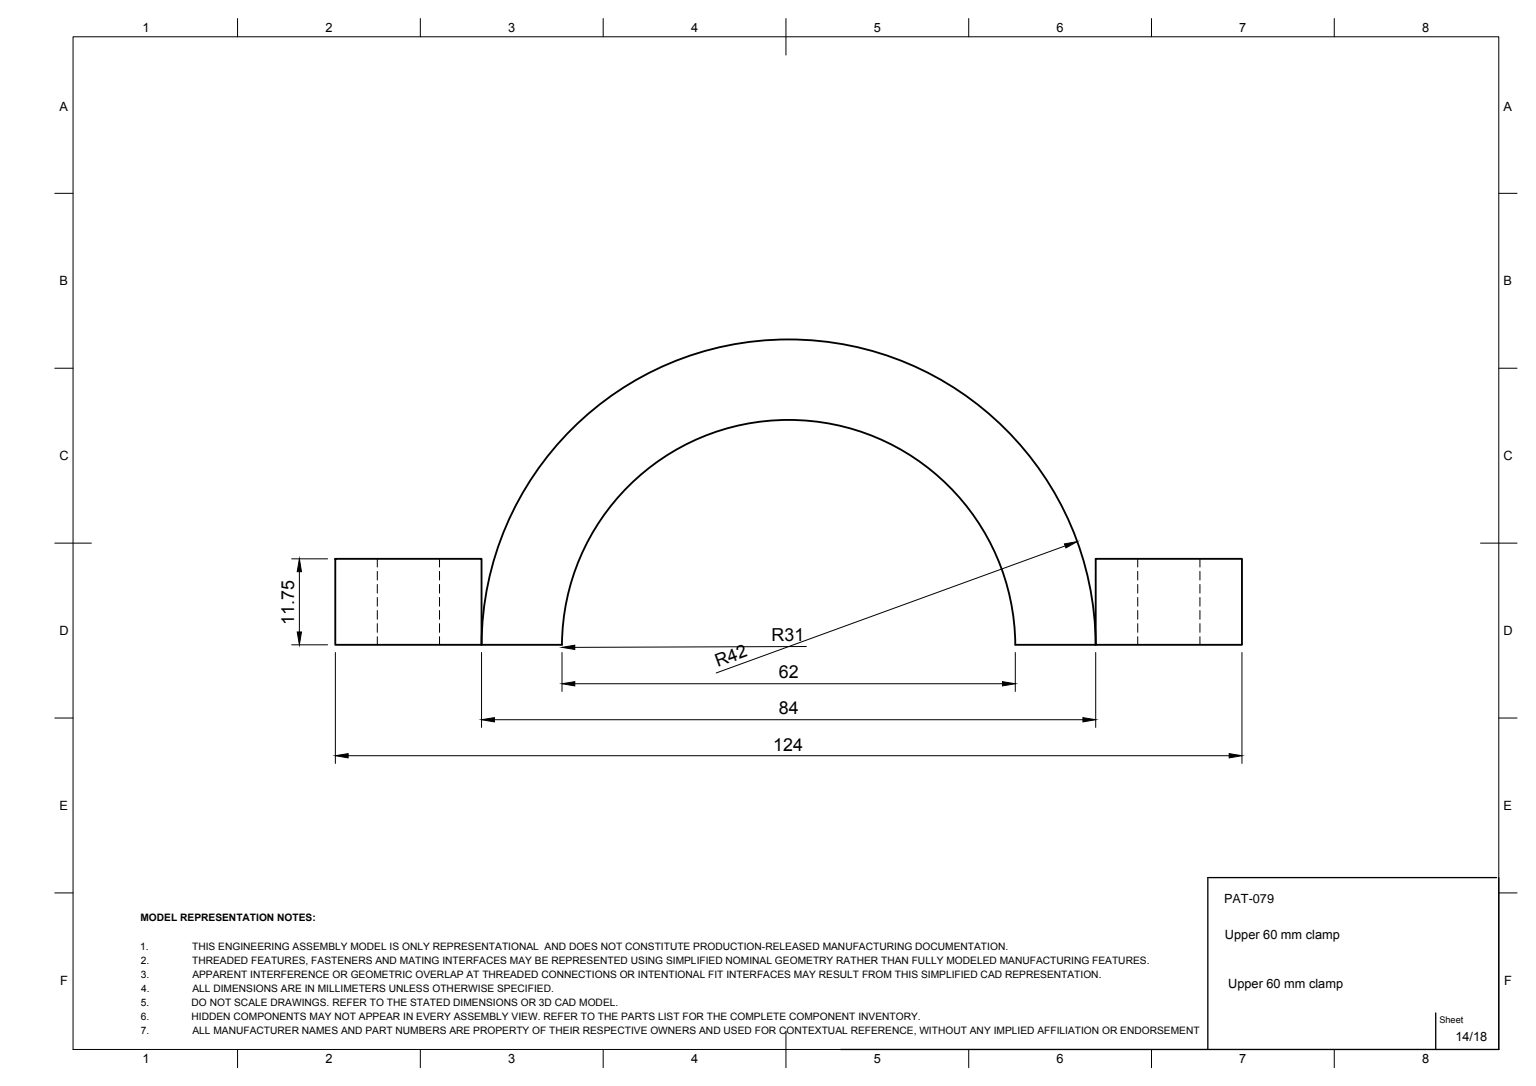
ISO-10303-21;
HEADER;
/* Generated by software containing ST-Developer
 * from STEP Tools, Inc. (www.steptools.com) 
 */

FILE_DESCRIPTION(
/* description */ ('Pipe clamp stand with threaded column'),
/* implementation_level */ '2;1');

FILE_NAME(
/* name */ 'Upper 60 mm clamp.step',
/* time_stamp */ '2026-10-27T10:55:48-07:00',
/* author */ (''),
/* organization */ (''),
/* preprocessor_version */ 'ST-DEVELOPER v20.2',
/* originating_system */ 'Autodesk Translation Framework v15.17.0.0',
/* authorisation */ '');

FILE_SCHEMA (('AUTOMOTIVE_DESIGN { 1 0 10303 214 3 1 1 }'));
ENDSEC;

DATA;
#10=MECHANICAL_DESIGN_GEOMETRIC_PRESENTATION_REPRESENTATION('',(#756,#757,#758),#34433);
#706=SHAPE_REPRESENTATION_RELATIONSHIP('SRR','None',#34548,#728);
#728=ADVANCED_BREP_SHAPE_REPRESENTATION('',(#786,#787,#788),#34416);
#756=STYLED_ITEM('',(#34729),#786);
#757=STYLED_ITEM('',(#34729),#787);
#758=STYLED_ITEM('',(#34729),#788);
#786=MANIFOLD_SOLID_BREP('Body1',#8783);
#787=MANIFOLD_SOLID_BREP('Body2',#8784);
#788=MANIFOLD_SOLID_BREP('Body3',#8785);
#838=FACE_BOUND('',#1893,.T.);
#839=FACE_BOUND('',#1896,.T.);
#840=FACE_BOUND('',#1902,.T.);
#841=FACE_BOUND('',#1905,.T.);
#943=PLANE('',#9448);
#944=PLANE('',#9450);
#945=PLANE('',#9451);
#946=PLANE('',#9454);
#947=PLANE('',#9458);
#948=PLANE('',#9459);
#949=PLANE('',#9460);
#950=PLANE('',#9461);
#951=PLANE('',#9462);
#952=PLANE('',#9463);
#953=PLANE('',#9467);
#954=PLANE('',#9468);
#955=PLANE('',#9469);
#956=PLANE('',#9470);
#957=PLANE('',#9471);
#958=PLANE('',#9472);
#1358=FACE_OUTER_BOUND('',#1884,.T.);
#1359=FACE_OUTER_BOUND('',#1885,.T.);
#1360=FACE_OUTER_BOUND('',#1886,.T.);
#1361=FACE_OUTER_BOUND('',#1887,.T.);
#1362=FACE_OUTER_BOUND('',#1888,.T.);
#1363=FACE_OUTER_BOUND('',#1889,.T.);
#1364=FACE_OUTER_BOUND('',#1890,.T.);
#1365=FACE_OUTER_BOUND('',#1891,.T.);
#1366=FACE_OUTER_BOUND('',#1892,.T.);
#1367=FACE_OUTER_BOUND('',#1894,.T.);
#1368=FACE_OUTER_BOUND('',#1895,.T.);
#1369=FACE_OUTER_BOUND('',#1897,.T.);
#1370=FACE_OUTER_BOUND('',#1898,.T.);
#1371=FACE_OUTER_BOUND('',#1899,.T.);
#1372=FACE_OUTER_BOUND('',#1900,.T.);
#1373=FACE_OUTER_BOUND('',#1901,.T.);
#1374=FACE_OUTER_BOUND('',#1903,.T.);
#1375=FACE_OUTER_BOUND('',#1904,.T.);
#1376=FACE_OUTER_BOUND('',#1906,.T.);
#1377=FACE_OUTER_BOUND('',#1907,.T.);
#1884=EDGE_LOOP('',(#7199,#7200,#7201,#7202));
#1885=EDGE_LOOP('',(#7203,#7204,#7205,#7206));
#1886=EDGE_LOOP('',(#7207,#7208,#7209,#7210));
#1887=EDGE_LOOP('',(#7211,#7212,#7213,#7214));
#1888=EDGE_LOOP('',(#7215,#7216,#7217,#7218));
#1889=EDGE_LOOP('',(#7219,#7220,#7221,#7222));
#1890=EDGE_LOOP('',(#7223,#7224,#7225,#7226));
#1891=EDGE_LOOP('',(#7227,#7228,#7229,#7230));
#1892=EDGE_LOOP('',(#7231,#7232,#7233,#7234));
#1893=EDGE_LOOP('',(#7235));
#1894=EDGE_LOOP('',(#7236,#7237,#7238,#7239));
#1895=EDGE_LOOP('',(#7240,#7241,#7242,#7243));
#1896=EDGE_LOOP('',(#7244));
#1897=EDGE_LOOP('',(#7245,#7246,#7247,#7248));
#1898=EDGE_LOOP('',(#7249,#7250,#7251,#7252));
#1899=EDGE_LOOP('',(#7253,#7254,#7255,#7256));
#1900=EDGE_LOOP('',(#7257,#7258,#7259,#7260));
#1901=EDGE_LOOP('',(#7261,#7262,#7263,#7264));
#1902=EDGE_LOOP('',(#7265));
#1903=EDGE_LOOP('',(#7266,#7267,#7268,#7269));
#1904=EDGE_LOOP('',(#7270,#7271,#7272,#7273));
#1905=EDGE_LOOP('',(#7274));
#1906=EDGE_LOOP('',(#7275,#7276,#7277,#7278));
#1907=EDGE_LOOP('',(#7279,#7280,#7281,#7282));
#2457=LINE('',#28483,#3074);
#2458=LINE('',#28487,#3075);
#2459=LINE('',#28491,#3076);
#2460=LINE('',#28494,#3077);
#2461=LINE('',#28497,#3078);
#2462=LINE('',#28498,#3079);
#2463=LINE('',#28501,#3080);
#2464=LINE('',#28502,#3081);
#2465=LINE('',#28510,#3082);
#2466=LINE('',#28515,#3083);
#2467=LINE('',#28517,#3084);
#2468=LINE('',#28519,#3085);
#2469=LINE('',#28520,#3086);
#2470=LINE('',#28523,#3087);
#2471=LINE('',#28525,#3088);
#2472=LINE('',#28526,#3089);
#2473=LINE('',#28529,#3090);
#2474=LINE('',#28531,#3091);
#2475=LINE('',#28532,#3092);
#2476=LINE('',#28534,#3093);
#2477=LINE('',#28535,#3094);
#2478=LINE('',#28542,#3095);
#2479=LINE('',#28547,#3096);
#2480=LINE('',#28549,#3097);
#2481=LINE('',#28551,#3098);
#2482=LINE('',#28552,#3099);
#2483=LINE('',#28555,#3100);
#2484=LINE('',#28557,#3101);
#2485=LINE('',#28558,#3102);
#2486=LINE('',#28561,#3103);
#2487=LINE('',#28563,#3104);
#2488=LINE('',#28564,#3105);
#2489=LINE('',#28566,#3106);
#2490=LINE('',#28567,#3107);
#3074=VECTOR('',#10912,1.);
#3075=VECTOR('',#10915,1.);
#3076=VECTOR('',#10920,1.);
#3077=VECTOR('',#10923,1.);
#3078=VECTOR('',#10926,1.);
#3079=VECTOR('',#10927,1.);
#3080=VECTOR('',#10930,1.);
#3081=VECTOR('',#10931,1.);
#3082=VECTOR('',#10942,0.425);
#3083=VECTOR('',#10947,1.);
#3084=VECTOR('',#10948,1.);
#3085=VECTOR('',#10949,1.);
#3086=VECTOR('',#10950,1.);
#3087=VECTOR('',#10953,1.);
#3088=VECTOR('',#10954,1.);
#3089=VECTOR('',#10955,1.);
#3090=VECTOR('',#10958,1.);
#3091=VECTOR('',#10959,1.);
#3092=VECTOR('',#10960,1.);
#3093=VECTOR('',#10963,1.);
#3094=VECTOR('',#10964,1.);
#3095=VECTOR('',#10973,0.425);
#3096=VECTOR('',#10978,1.);
#3097=VECTOR('',#10979,1.);
#3098=VECTOR('',#10980,1.);
#3099=VECTOR('',#10981,1.);
#3100=VECTOR('',#10984,1.);
#3101=VECTOR('',#10985,1.);
#3102=VECTOR('',#10986,1.);
#3103=VECTOR('',#10989,1.);
#3104=VECTOR('',#10990,1.);
#3105=VECTOR('',#10991,1.);
#3106=VECTOR('',#10994,1.);
#3107=VECTOR('',#10995,1.);
#3388=CIRCLE('',#9446,3.1);
#3389=CIRCLE('',#9447,3.1);
#3390=CIRCLE('',#9449,4.2);
#3391=CIRCLE('',#9453,4.2);
#3392=CIRCLE('',#9456,0.425);
#3393=CIRCLE('',#9457,0.425);
#3394=CIRCLE('',#9465,0.425);
#3395=CIRCLE('',#9466,0.425);
#4006=VERTEX_POINT('',#28481);
#4007=VERTEX_POINT('',#28482);
#4008=VERTEX_POINT('',#28484);
#4009=VERTEX_POINT('',#28486);
#4010=VERTEX_POINT('',#28490);
#4011=VERTEX_POINT('',#28492);
#4012=VERTEX_POINT('',#28496);
#4013=VERTEX_POINT('',#28500);
#4014=VERTEX_POINT('',#28507);
#4015=VERTEX_POINT('',#28509);
#4016=VERTEX_POINT('',#28513);
#4017=VERTEX_POINT('',#28514);
#4018=VERTEX_POINT('',#28516);
#4019=VERTEX_POINT('',#28518);
#4020=VERTEX_POINT('',#28522);
#4021=VERTEX_POINT('',#28524);
#4022=VERTEX_POINT('',#28528);
#4023=VERTEX_POINT('',#28530);
#4024=VERTEX_POINT('',#28539);
#4025=VERTEX_POINT('',#28541);
#4026=VERTEX_POINT('',#28545);
#4027=VERTEX_POINT('',#28546);
#4028=VERTEX_POINT('',#28548);
#4029=VERTEX_POINT('',#28550);
#4030=VERTEX_POINT('',#28554);
#4031=VERTEX_POINT('',#28556);
#4032=VERTEX_POINT('',#28560);
#4033=VERTEX_POINT('',#28562);
#5113=EDGE_CURVE('',#4006,#4007,#2457,.T.);
#5114=EDGE_CURVE('',#4008,#4006,#3388,.T.);
#5115=EDGE_CURVE('',#4009,#4008,#2458,.T.);
#5116=EDGE_CURVE('',#4007,#4009,#3389,.T.);
#5117=EDGE_CURVE('',#4006,#4010,#2459,.T.);
#5118=EDGE_CURVE('',#4010,#4011,#3390,.T.);
#5119=EDGE_CURVE('',#4011,#4008,#2460,.T.);
#5120=EDGE_CURVE('',#4012,#4007,#2461,.T.);
#5121=EDGE_CURVE('',#4010,#4012,#2462,.T.);
#5122=EDGE_CURVE('',#4013,#4011,#2463,.T.);
#5123=EDGE_CURVE('',#4009,#4013,#2464,.T.);
#5124=EDGE_CURVE('',#4012,#4013,#3391,.T.);
#5125=EDGE_CURVE('',#4014,#4014,#3392,.T.);
#5126=EDGE_CURVE('',#4014,#4015,#2465,.T.);
#5127=EDGE_CURVE('',#4015,#4015,#3393,.T.);
#5128=EDGE_CURVE('',#4016,#4017,#2466,.T.);
#5129=EDGE_CURVE('',#4016,#4018,#2467,.T.);
#5130=EDGE_CURVE('',#4019,#4018,#2468,.T.);
#5131=EDGE_CURVE('',#4017,#4019,#2469,.T.);
#5132=EDGE_CURVE('',#4017,#4020,#2470,.T.);
#5133=EDGE_CURVE('',#4021,#4019,#2471,.T.);
#5134=EDGE_CURVE('',#4020,#4021,#2472,.T.);
#5135=EDGE_CURVE('',#4020,#4022,#2473,.T.);
#5136=EDGE_CURVE('',#4023,#4021,#2474,.T.);
#5137=EDGE_CURVE('',#4022,#4023,#2475,.T.);
#5138=EDGE_CURVE('',#4022,#4016,#2476,.T.);
#5139=EDGE_CURVE('',#4018,#4023,#2477,.T.);
#5140=EDGE_CURVE('',#4024,#4024,#3394,.T.);
#5141=EDGE_CURVE('',#4024,#4025,#2478,.T.);
#5142=EDGE_CURVE('',#4025,#4025,#3395,.T.);
#5143=EDGE_CURVE('',#4026,#4027,#2479,.T.);
#5144=EDGE_CURVE('',#4026,#4028,#2480,.T.);
#5145=EDGE_CURVE('',#4029,#4028,#2481,.T.);
#5146=EDGE_CURVE('',#4027,#4029,#2482,.T.);
#5147=EDGE_CURVE('',#4027,#4030,#2483,.T.);
#5148=EDGE_CURVE('',#4031,#4029,#2484,.T.);
#5149=EDGE_CURVE('',#4030,#4031,#2485,.T.);
#5150=EDGE_CURVE('',#4030,#4032,#2486,.T.);
#5151=EDGE_CURVE('',#4033,#4031,#2487,.T.);
#5152=EDGE_CURVE('',#4032,#4033,#2488,.T.);
#5153=EDGE_CURVE('',#4032,#4026,#2489,.T.);
#5154=EDGE_CURVE('',#4028,#4033,#2490,.T.);
#7199=ORIENTED_EDGE('',*,*,#5113,.F.);
#7200=ORIENTED_EDGE('',*,*,#5114,.F.);
#7201=ORIENTED_EDGE('',*,*,#5115,.F.);
#7202=ORIENTED_EDGE('',*,*,#5116,.F.);
#7203=ORIENTED_EDGE('',*,*,#5114,.T.);
#7204=ORIENTED_EDGE('',*,*,#5117,.T.);
#7205=ORIENTED_EDGE('',*,*,#5118,.T.);
#7206=ORIENTED_EDGE('',*,*,#5119,.T.);
#7207=ORIENTED_EDGE('',*,*,#5113,.T.);
#7208=ORIENTED_EDGE('',*,*,#5120,.F.);
#7209=ORIENTED_EDGE('',*,*,#5121,.F.);
#7210=ORIENTED_EDGE('',*,*,#5117,.F.);
#7211=ORIENTED_EDGE('',*,*,#5115,.T.);
#7212=ORIENTED_EDGE('',*,*,#5119,.F.);
#7213=ORIENTED_EDGE('',*,*,#5122,.F.);
#7214=ORIENTED_EDGE('',*,*,#5123,.F.);
#7215=ORIENTED_EDGE('',*,*,#5122,.T.);
#7216=ORIENTED_EDGE('',*,*,#5118,.F.);
#7217=ORIENTED_EDGE('',*,*,#5121,.T.);
#7218=ORIENTED_EDGE('',*,*,#5124,.T.);
#7219=ORIENTED_EDGE('',*,*,#5116,.T.);
#7220=ORIENTED_EDGE('',*,*,#5123,.T.);
#7221=ORIENTED_EDGE('',*,*,#5124,.F.);
#7222=ORIENTED_EDGE('',*,*,#5120,.T.);
#7223=ORIENTED_EDGE('',*,*,#5125,.F.);
#7224=ORIENTED_EDGE('',*,*,#5126,.T.);
#7225=ORIENTED_EDGE('',*,*,#5127,.F.);
#7226=ORIENTED_EDGE('',*,*,#5126,.F.);
#7227=ORIENTED_EDGE('',*,*,#5128,.F.);
#7228=ORIENTED_EDGE('',*,*,#5129,.T.);
#7229=ORIENTED_EDGE('',*,*,#5130,.F.);
#7230=ORIENTED_EDGE('',*,*,#5131,.F.);
#7231=ORIENTED_EDGE('',*,*,#5132,.F.);
#7232=ORIENTED_EDGE('',*,*,#5131,.T.);
#7233=ORIENTED_EDGE('',*,*,#5133,.F.);
#7234=ORIENTED_EDGE('',*,*,#5134,.F.);
#7235=ORIENTED_EDGE('',*,*,#5125,.T.);
#7236=ORIENTED_EDGE('',*,*,#5135,.F.);
#7237=ORIENTED_EDGE('',*,*,#5134,.T.);
#7238=ORIENTED_EDGE('',*,*,#5136,.F.);
#7239=ORIENTED_EDGE('',*,*,#5137,.F.);
#7240=ORIENTED_EDGE('',*,*,#5138,.F.);
#7241=ORIENTED_EDGE('',*,*,#5137,.T.);
#7242=ORIENTED_EDGE('',*,*,#5139,.F.);
#7243=ORIENTED_EDGE('',*,*,#5129,.F.);
#7244=ORIENTED_EDGE('',*,*,#5127,.T.);
#7245=ORIENTED_EDGE('',*,*,#5139,.T.);
#7246=ORIENTED_EDGE('',*,*,#5136,.T.);
#7247=ORIENTED_EDGE('',*,*,#5133,.T.);
#7248=ORIENTED_EDGE('',*,*,#5130,.T.);
#7249=ORIENTED_EDGE('',*,*,#5138,.T.);
#7250=ORIENTED_EDGE('',*,*,#5128,.T.);
#7251=ORIENTED_EDGE('',*,*,#5132,.T.);
#7252=ORIENTED_EDGE('',*,*,#5135,.T.);
#7253=ORIENTED_EDGE('',*,*,#5140,.F.);
#7254=ORIENTED_EDGE('',*,*,#5141,.T.);
#7255=ORIENTED_EDGE('',*,*,#5142,.F.);
#7256=ORIENTED_EDGE('',*,*,#5141,.F.);
#7257=ORIENTED_EDGE('',*,*,#5143,.F.);
#7258=ORIENTED_EDGE('',*,*,#5144,.T.);
#7259=ORIENTED_EDGE('',*,*,#5145,.F.);
#7260=ORIENTED_EDGE('',*,*,#5146,.F.);
#7261=ORIENTED_EDGE('',*,*,#5147,.F.);
#7262=ORIENTED_EDGE('',*,*,#5146,.T.);
#7263=ORIENTED_EDGE('',*,*,#5148,.F.);
#7264=ORIENTED_EDGE('',*,*,#5149,.F.);
#7265=ORIENTED_EDGE('',*,*,#5140,.T.);
#7266=ORIENTED_EDGE('',*,*,#5150,.F.);
#7267=ORIENTED_EDGE('',*,*,#5149,.T.);
#7268=ORIENTED_EDGE('',*,*,#5151,.F.);
#7269=ORIENTED_EDGE('',*,*,#5152,.F.);
#7270=ORIENTED_EDGE('',*,*,#5153,.F.);
#7271=ORIENTED_EDGE('',*,*,#5152,.T.);
#7272=ORIENTED_EDGE('',*,*,#5154,.F.);
#7273=ORIENTED_EDGE('',*,*,#5144,.F.);
#7274=ORIENTED_EDGE('',*,*,#5142,.T.);
#7275=ORIENTED_EDGE('',*,*,#5154,.T.);
#7276=ORIENTED_EDGE('',*,*,#5151,.T.);
#7277=ORIENTED_EDGE('',*,*,#5148,.T.);
#7278=ORIENTED_EDGE('',*,*,#5145,.T.);
#7279=ORIENTED_EDGE('',*,*,#5153,.T.);
#7280=ORIENTED_EDGE('',*,*,#5143,.T.);
#7281=ORIENTED_EDGE('',*,*,#5147,.T.);
#7282=ORIENTED_EDGE('',*,*,#5150,.T.);
#8225=CYLINDRICAL_SURFACE('',#9445,3.1);
#8226=CYLINDRICAL_SURFACE('',#9452,4.2);
#8227=CYLINDRICAL_SURFACE('',#9455,0.425);
#8228=CYLINDRICAL_SURFACE('',#9464,0.425);
#8595=ADVANCED_FACE('',(#1358),#8225,.F.);
#8596=ADVANCED_FACE('',(#1359),#943,.T.);
#8597=ADVANCED_FACE('',(#1360),#944,.F.);
#8598=ADVANCED_FACE('',(#1361),#945,.F.);
#8599=ADVANCED_FACE('',(#1362),#8226,.T.);
#8600=ADVANCED_FACE('',(#1363),#946,.F.);
#8601=ADVANCED_FACE('',(#1364),#8227,.F.);
#8602=ADVANCED_FACE('',(#1365),#947,.T.);
#8603=ADVANCED_FACE('',(#1366,#838),#948,.T.);
#8604=ADVANCED_FACE('',(#1367),#949,.T.);
#8605=ADVANCED_FACE('',(#1368,#839),#950,.T.);
#8606=ADVANCED_FACE('',(#1369),#951,.T.);
#8607=ADVANCED_FACE('',(#1370),#952,.F.);
#8608=ADVANCED_FACE('',(#1371),#8228,.F.);
#8609=ADVANCED_FACE('',(#1372),#953,.T.);
#8610=ADVANCED_FACE('',(#1373,#840),#954,.T.);
#8611=ADVANCED_FACE('',(#1374),#955,.T.);
#8612=ADVANCED_FACE('',(#1375,#841),#956,.T.);
#8613=ADVANCED_FACE('',(#1376),#957,.T.);
#8614=ADVANCED_FACE('',(#1377),#958,.F.);
#8783=CLOSED_SHELL('',(#8595,#8596,#8597,#8598,#8599,#8600));
#8784=CLOSED_SHELL('',(#8601,#8602,#8603,#8604,#8605,#8606,#8607));
#8785=CLOSED_SHELL('',(#8608,#8609,#8610,#8611,#8612,#8613,#8614));
#9444=AXIS2_PLACEMENT_3D('',#28479,#10908,#10909);
#9445=AXIS2_PLACEMENT_3D('',#28480,#10910,#10911);
#9446=AXIS2_PLACEMENT_3D('',#28485,#10913,#10914);
#9447=AXIS2_PLACEMENT_3D('',#28488,#10916,#10917);
#9448=AXIS2_PLACEMENT_3D('',#28489,#10918,#10919);
#9449=AXIS2_PLACEMENT_3D('',#28493,#10921,#10922);
#9450=AXIS2_PLACEMENT_3D('',#28495,#10924,#10925);
#9451=AXIS2_PLACEMENT_3D('',#28499,#10928,#10929);
#9452=AXIS2_PLACEMENT_3D('',#28503,#10932,#10933);
#9453=AXIS2_PLACEMENT_3D('',#28504,#10934,#10935);
#9454=AXIS2_PLACEMENT_3D('',#28505,#10936,#10937);
#9455=AXIS2_PLACEMENT_3D('',#28506,#10938,#10939);
#9456=AXIS2_PLACEMENT_3D('',#28508,#10940,#10941);
#9457=AXIS2_PLACEMENT_3D('',#28511,#10943,#10944);
#9458=AXIS2_PLACEMENT_3D('',#28512,#10945,#10946);
#9459=AXIS2_PLACEMENT_3D('',#28521,#10951,#10952);
#9460=AXIS2_PLACEMENT_3D('',#28527,#10956,#10957);
#9461=AXIS2_PLACEMENT_3D('',#28533,#10961,#10962);
#9462=AXIS2_PLACEMENT_3D('',#28536,#10965,#10966);
#9463=AXIS2_PLACEMENT_3D('',#28537,#10967,#10968);
#9464=AXIS2_PLACEMENT_3D('',#28538,#10969,#10970);
#9465=AXIS2_PLACEMENT_3D('',#28540,#10971,#10972);
#9466=AXIS2_PLACEMENT_3D('',#28543,#10974,#10975);
#9467=AXIS2_PLACEMENT_3D('',#28544,#10976,#10977);
#9468=AXIS2_PLACEMENT_3D('',#28553,#10982,#10983);
#9469=AXIS2_PLACEMENT_3D('',#28559,#10987,#10988);
#9470=AXIS2_PLACEMENT_3D('',#28565,#10992,#10993);
#9471=AXIS2_PLACEMENT_3D('',#28568,#10996,#10997);
#9472=AXIS2_PLACEMENT_3D('',#28569,#10998,#10999);
#10908=DIRECTION('axis',(0.,0.,1.));
#10909=DIRECTION('refdir',(1.,0.,0.));
#10910=DIRECTION('center_axis',(0.,1.,0.));
#10911=DIRECTION('ref_axis',(1.,0.,0.));
#10912=DIRECTION('',(0.,-1.,0.));
#10913=DIRECTION('center_axis',(0.,-1.,0.));
#10914=DIRECTION('ref_axis',(1.,0.,0.));
#10915=DIRECTION('',(0.,1.,0.));
#10916=DIRECTION('center_axis',(0.,1.,0.));
#10917=DIRECTION('ref_axis',(1.,0.,0.));
#10918=DIRECTION('center_axis',(0.,1.,0.));
#10919=DIRECTION('ref_axis',(1.,0.,0.));
#10920=DIRECTION('',(-1.,0.,0.));
#10921=DIRECTION('center_axis',(0.,1.,0.));
#10922=DIRECTION('ref_axis',(1.,0.,0.));
#10923=DIRECTION('',(-1.,0.,0.));
#10924=DIRECTION('center_axis',(0.,0.,1.));
#10925=DIRECTION('ref_axis',(1.,0.,0.));
#10926=DIRECTION('',(1.,0.,0.));
#10927=DIRECTION('',(0.,-1.,0.));
#10928=DIRECTION('center_axis',(0.,0.,1.));
#10929=DIRECTION('ref_axis',(1.,0.,0.));
#10930=DIRECTION('',(0.,1.,0.));
#10931=DIRECTION('',(1.,0.,0.));
#10932=DIRECTION('center_axis',(0.,1.,0.));
#10933=DIRECTION('ref_axis',(1.,0.,0.));
#10934=DIRECTION('center_axis',(0.,1.,0.));
#10935=DIRECTION('ref_axis',(1.,0.,0.));
#10936=DIRECTION('center_axis',(0.,1.,0.));
#10937=DIRECTION('ref_axis',(1.,0.,0.));
#10938=DIRECTION('center_axis',(0.,0.,1.));
#10939=DIRECTION('ref_axis',(1.,0.,0.));
#10940=DIRECTION('center_axis',(0.,0.,1.));
#10941=DIRECTION('ref_axis',(1.,0.,0.));
#10942=DIRECTION('',(0.,0.,1.));
#10943=DIRECTION('center_axis',(0.,0.,-1.));
#10944=DIRECTION('ref_axis',(1.,0.,0.));
#10945=DIRECTION('center_axis',(-1.,0.,0.));
#10946=DIRECTION('ref_axis',(0.,0.,1.));
#10947=DIRECTION('',(0.,0.,-1.));
#10948=DIRECTION('',(0.,1.,0.));
#10949=DIRECTION('',(0.,0.,1.));
#10950=DIRECTION('',(0.,1.,0.));
#10951=DIRECTION('center_axis',(0.,0.,-1.));
#10952=DIRECTION('ref_axis',(-1.,0.,0.));
#10953=DIRECTION('',(1.,0.,0.));
#10954=DIRECTION('',(-1.,0.,0.));
#10955=DIRECTION('',(0.,1.,0.));
#10956=DIRECTION('center_axis',(1.,0.,0.));
#10957=DIRECTION('ref_axis',(0.,0.,-1.));
#10958=DIRECTION('',(0.,0.,1.));
#10959=DIRECTION('',(0.,0.,-1.));
#10960=DIRECTION('',(0.,1.,0.));
#10961=DIRECTION('center_axis',(0.,0.,1.));
#10962=DIRECTION('ref_axis',(1.,0.,0.));
#10963=DIRECTION('',(-1.,0.,0.));
#10964=DIRECTION('',(1.,0.,0.));
#10965=DIRECTION('center_axis',(0.,1.,0.));
#10966=DIRECTION('ref_axis',(0.,0.,1.));
#10967=DIRECTION('center_axis',(0.,1.,0.));
#10968=DIRECTION('ref_axis',(1.,0.,0.));
#10969=DIRECTION('center_axis',(0.,0.,1.));
#10970=DIRECTION('ref_axis',(1.,0.,0.));
#10971=DIRECTION('center_axis',(0.,0.,1.));
#10972=DIRECTION('ref_axis',(1.,0.,0.));
#10973=DIRECTION('',(0.,0.,1.));
#10974=DIRECTION('center_axis',(0.,0.,-1.));
#10975=DIRECTION('ref_axis',(1.,0.,0.));
#10976=DIRECTION('center_axis',(-1.,0.,0.));
#10977=DIRECTION('ref_axis',(0.,0.,1.));
#10978=DIRECTION('',(0.,0.,-1.));
#10979=DIRECTION('',(0.,1.,0.));
#10980=DIRECTION('',(0.,0.,1.));
#10981=DIRECTION('',(0.,1.,0.));
#10982=DIRECTION('center_axis',(0.,0.,-1.));
#10983=DIRECTION('ref_axis',(-1.,0.,0.));
#10984=DIRECTION('',(1.,0.,0.));
#10985=DIRECTION('',(-1.,0.,0.));
#10986=DIRECTION('',(0.,1.,0.));
#10987=DIRECTION('center_axis',(1.,0.,0.));
#10988=DIRECTION('ref_axis',(0.,0.,-1.));
#10989=DIRECTION('',(0.,0.,1.));
#10990=DIRECTION('',(0.,0.,-1.));
#10991=DIRECTION('',(0.,1.,0.));
#10992=DIRECTION('center_axis',(0.,0.,1.));
#10993=DIRECTION('ref_axis',(1.,0.,0.));
#10994=DIRECTION('',(-1.,0.,0.));
#10995=DIRECTION('',(1.,0.,0.));
#10996=DIRECTION('center_axis',(0.,1.,0.));
#10997=DIRECTION('ref_axis',(0.,0.,1.));
#10998=DIRECTION('center_axis',(0.,1.,0.));
#10999=DIRECTION('ref_axis',(1.,0.,0.));
#28479=CARTESIAN_POINT('',(0.,0.,0.));
#28480=CARTESIAN_POINT('Origin',(0.,-1.1,28.));
#28481=CARTESIAN_POINT('',(-3.09989919190931,1.,28.025));
#28482=CARTESIAN_POINT('',(-3.09989919190931,-1.,28.025));
#28483=CARTESIAN_POINT('',(-3.09989919190931,-1.1,28.025));
#28484=CARTESIAN_POINT('',(3.09989919190931,1.,28.025));
#28485=CARTESIAN_POINT('Origin',(0.,1.,28.));
#28486=CARTESIAN_POINT('',(3.09989919190931,-1.,28.025));
#28487=CARTESIAN_POINT('',(3.09989919190931,-1.1,28.025));
#28488=CARTESIAN_POINT('Origin',(0.,-1.,28.));
#28489=CARTESIAN_POINT('Origin',(0.,1.,28.));
#28490=CARTESIAN_POINT('',(-4.19992559457903,1.,28.025));
#28491=CARTESIAN_POINT('',(-4.2,1.,28.025));
#28492=CARTESIAN_POINT('',(4.19992559457903,1.,28.025));
#28493=CARTESIAN_POINT('Origin',(0.,1.,28.));
#28494=CARTESIAN_POINT('',(-4.2,1.,28.025));
#28495=CARTESIAN_POINT('Origin',(-8.4,-1.1,28.025));
#28496=CARTESIAN_POINT('',(-4.19992559457903,-1.,28.025));
#28497=CARTESIAN_POINT('',(-4.2,-1.,28.025));
#28498=CARTESIAN_POINT('',(-4.19992559457903,-1.,28.025));
#28499=CARTESIAN_POINT('Origin',(-8.4,-1.1,28.025));
#28500=CARTESIAN_POINT('',(4.19992559457903,-1.,28.025));
#28501=CARTESIAN_POINT('',(4.19992559457903,-1.,28.025));
#28502=CARTESIAN_POINT('',(-4.2,-1.,28.025));
#28503=CARTESIAN_POINT('Origin',(0.,-1.,28.));
#28504=CARTESIAN_POINT('Origin',(0.,-1.,28.));
#28505=CARTESIAN_POINT('Origin',(0.,-1.,28.));
#28506=CARTESIAN_POINT('Origin',(-5.2,0.,26.7));
#28507=CARTESIAN_POINT('',(-5.625,-5.20474889637625E-17,28.025));
#28508=CARTESIAN_POINT('Origin',(-5.2,0.,28.025));
#28509=CARTESIAN_POINT('',(-5.625,5.20474889637625E-17,29.2));
#28510=CARTESIAN_POINT('',(-5.625,-5.20474889637625E-17,26.7));
#28511=CARTESIAN_POINT('Origin',(-5.2,0.,29.2));
#28512=CARTESIAN_POINT('Origin',(-6.2,-1.,28.025));
#28513=CARTESIAN_POINT('',(-6.2,-1.,29.2));
#28514=CARTESIAN_POINT('',(-6.2,-1.,28.025));
#28515=CARTESIAN_POINT('',(-6.2,-1.,29.2));
#28516=CARTESIAN_POINT('',(-6.2,1.,29.2));
#28517=CARTESIAN_POINT('',(-6.2,-1.,29.2));
#28518=CARTESIAN_POINT('',(-6.2,1.,28.025));
#28519=CARTESIAN_POINT('',(-6.2,1.,29.2));
#28520=CARTESIAN_POINT('',(-6.2,-1.,28.025));
#28521=CARTESIAN_POINT('Origin',(-4.2,-1.,28.025));
#28522=CARTESIAN_POINT('',(-4.2,-1.,28.025));
#28523=CARTESIAN_POINT('',(-6.2,-1.,28.025));
#28524=CARTESIAN_POINT('',(-4.2,1.,28.025));
#28525=CARTESIAN_POINT('',(-6.2,1.,28.025));
#28526=CARTESIAN_POINT('',(-4.2,-1.,28.025));
#28527=CARTESIAN_POINT('Origin',(-4.2,-1.,29.2));
#28528=CARTESIAN_POINT('',(-4.2,-1.,29.2));
#28529=CARTESIAN_POINT('',(-4.2,-1.,28.025));
#28530=CARTESIAN_POINT('',(-4.2,1.,29.2));
#28531=CARTESIAN_POINT('',(-4.2,1.,28.025));
#28532=CARTESIAN_POINT('',(-4.2,-1.,29.2));
#28533=CARTESIAN_POINT('Origin',(-6.2,-1.,29.2));
#28534=CARTESIAN_POINT('',(-4.2,-1.,29.2));
#28535=CARTESIAN_POINT('',(-4.2,1.,29.2));
#28536=CARTESIAN_POINT('Origin',(-5.2,1.,28.6125));
#28537=CARTESIAN_POINT('Origin',(-5.2,-1.,28.6125));
#28538=CARTESIAN_POINT('Origin',(5.2,0.,26.7));
#28539=CARTESIAN_POINT('',(4.775,-5.20474889637625E-17,28.025));
#28540=CARTESIAN_POINT('Origin',(5.2,0.,28.025));
#28541=CARTESIAN_POINT('',(4.775,5.20474889637625E-17,29.2));
#28542=CARTESIAN_POINT('',(4.775,-5.20474889637625E-17,26.7));
#28543=CARTESIAN_POINT('Origin',(5.2,0.,29.2));
#28544=CARTESIAN_POINT('Origin',(4.2,-1.,28.025));
#28545=CARTESIAN_POINT('',(4.2,-1.,29.2));
#28546=CARTESIAN_POINT('',(4.2,-1.,28.025));
#28547=CARTESIAN_POINT('',(4.2,-1.,29.2));
#28548=CARTESIAN_POINT('',(4.2,1.,29.2));
#28549=CARTESIAN_POINT('',(4.2,-1.,29.2));
#28550=CARTESIAN_POINT('',(4.2,1.,28.025));
#28551=CARTESIAN_POINT('',(4.2,1.,29.2));
#28552=CARTESIAN_POINT('',(4.2,-1.,28.025));
#28553=CARTESIAN_POINT('Origin',(6.2,-1.,28.025));
#28554=CARTESIAN_POINT('',(6.2,-1.,28.025));
#28555=CARTESIAN_POINT('',(4.2,-1.,28.025));
#28556=CARTESIAN_POINT('',(6.2,1.,28.025));
#28557=CARTESIAN_POINT('',(4.2,1.,28.025));
#28558=CARTESIAN_POINT('',(6.2,-1.,28.025));
#28559=CARTESIAN_POINT('Origin',(6.2,-1.,29.2));
#28560=CARTESIAN_POINT('',(6.2,-1.,29.2));
#28561=CARTESIAN_POINT('',(6.2,-1.,28.025));
#28562=CARTESIAN_POINT('',(6.2,1.,29.2));
#28563=CARTESIAN_POINT('',(6.2,1.,28.025));
#28564=CARTESIAN_POINT('',(6.2,-1.,29.2));
#28565=CARTESIAN_POINT('Origin',(4.2,-1.,29.2));
#28566=CARTESIAN_POINT('',(6.2,-1.,29.2));
#28567=CARTESIAN_POINT('',(6.2,1.,29.2));
#28568=CARTESIAN_POINT('Origin',(5.2,1.,28.6125));
#28569=CARTESIAN_POINT('Origin',(5.2,-1.,28.6125));
#34387=UNCERTAINTY_MEASURE_WITH_UNIT(LENGTH_MEASURE(0.001),#34434,
'DISTANCE_ACCURACY_VALUE',
'Maximum model space distance between geometric entities at asserted c
onnectivities');
#34404=UNCERTAINTY_MEASURE_WITH_UNIT(LENGTH_MEASURE(0.001),#34434,
'DISTANCE_ACCURACY_VALUE',
'Maximum model space distance between geometric entities at asserted c
onnectivities');
#34416=(
GEOMETRIC_REPRESENTATION_CONTEXT(3)
GLOBAL_UNCERTAINTY_ASSIGNED_CONTEXT((#34387))
GLOBAL_UNIT_ASSIGNED_CONTEXT((#34434,#34436,#34437))
REPRESENTATION_CONTEXT('','3D')
);
#34433=(
GEOMETRIC_REPRESENTATION_CONTEXT(3)
GLOBAL_UNCERTAINTY_ASSIGNED_CONTEXT((#34404))
GLOBAL_UNIT_ASSIGNED_CONTEXT((#34434,#34436,#34437))
REPRESENTATION_CONTEXT('','3D')
);
#34434=(
LENGTH_UNIT()
NAMED_UNIT(*)
SI_UNIT(.CENTI.,.METRE.)
);
#34436=(
NAMED_UNIT(*)
PLANE_ANGLE_UNIT()
SI_UNIT($,.RADIAN.)
);
#34437=(
NAMED_UNIT(*)
SI_UNIT($,.STERADIAN.)
SOLID_ANGLE_UNIT()
);
#34449=SHAPE_DEFINITION_REPRESENTATION(#34477,#34548);
#34477=PRODUCT_DEFINITION_SHAPE('',$,#34577);
#34548=SHAPE_REPRESENTATION('',(#9444),#34416);
#34565=PRODUCT_DEFINITION_CONTEXT('part definition',#34651,'design');
#34577=PRODUCT_DEFINITION('Upper 60 mm clamp','Upper 60 mm clamp',#34605,
#34565);
#34605=PRODUCT_DEFINITION_FORMATION('',$,#34664);
#34651=APPLICATION_CONTEXT(
'Core Data for Automotive Mechanical Design Process');
#34652=PRODUCT_CONTEXT('part definition',#34651,'mechanical');
#34664=PRODUCT('Upper 60 mm clamp','Upper 60 mm clamp',
'Upper 60 mm clamp',(#34652));
#34723=COLOUR_RGB('Light Blue',0.38,0.62,0.78);
#34724=FILL_AREA_STYLE_COLOUR('',#34723);
#34725=FILL_AREA_STYLE('',(#34724));
#34726=SURFACE_STYLE_FILL_AREA(#34725);
#34727=SURFACE_SIDE_STYLE('',(#34726));
#34728=SURFACE_STYLE_USAGE(.BOTH.,#34727);
#34729=PRESENTATION_STYLE_ASSIGNMENT((#34728));
ENDSEC;
END-ISO-10303-21;
